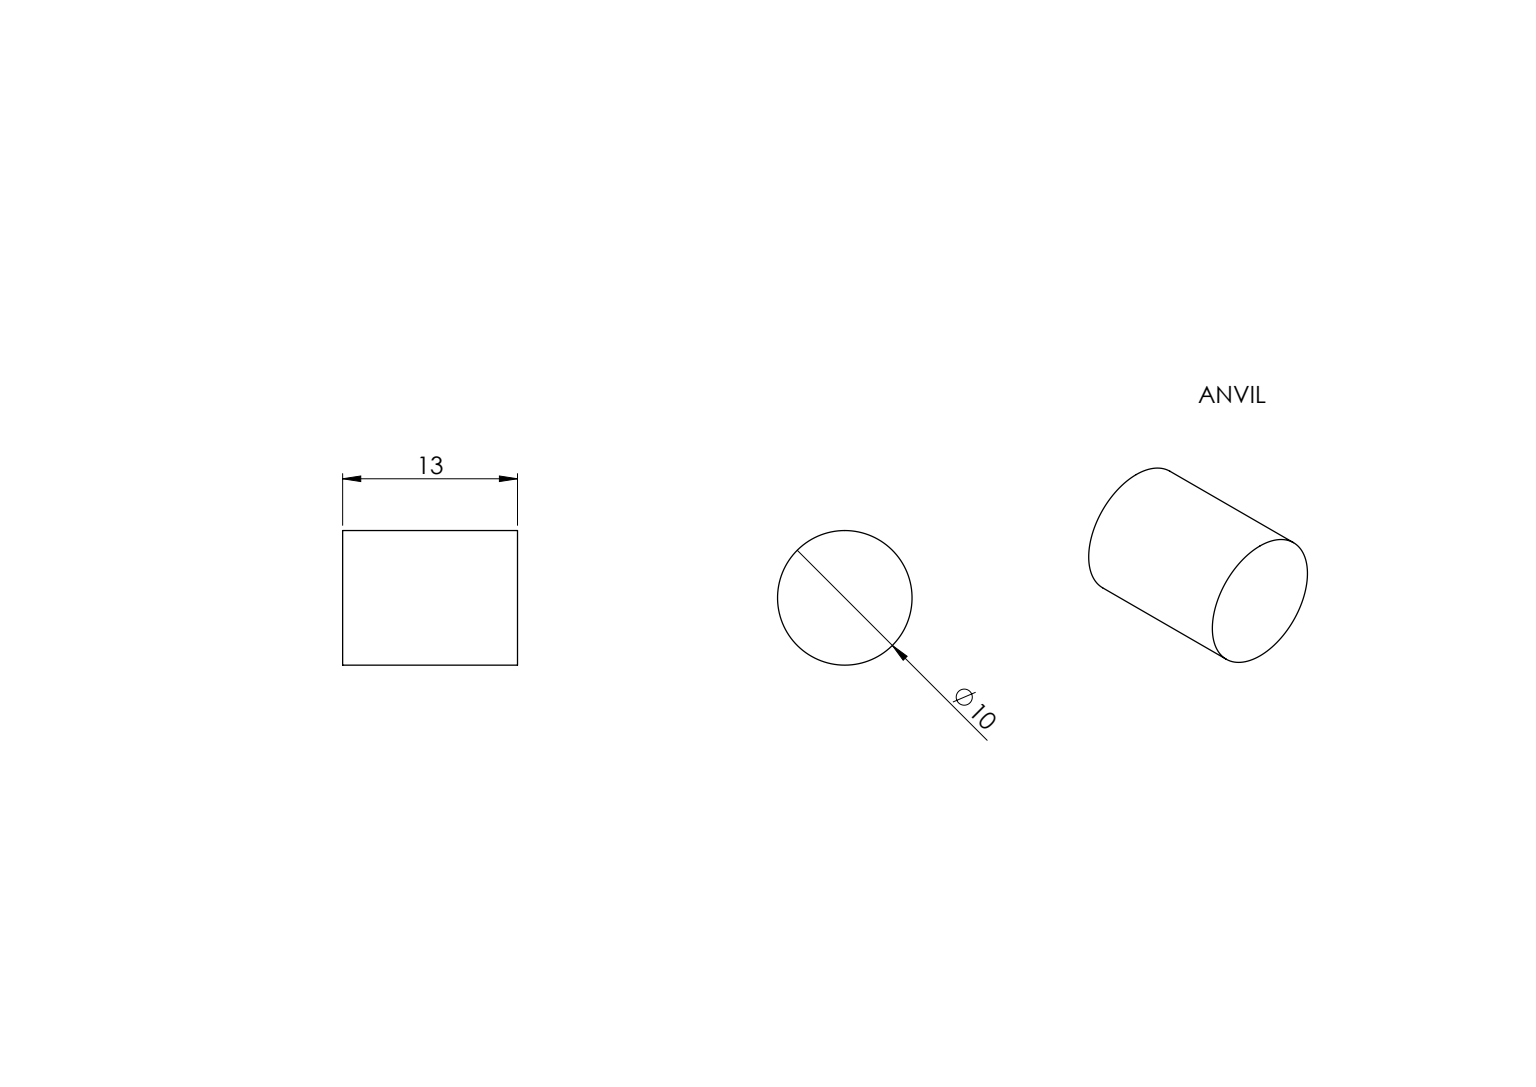
ISO-10303-21;
HEADER;
FILE_DESCRIPTION (('STEP AP214'),
    '1' );
FILE_NAME ('anvil.step',
    '2026-10-22T12:35:56',
    ( '' ),
    ( '' ),
    'SwSTEP 2.0',
    'SolidWorks 2026',
    '' );
FILE_SCHEMA (( 'AUTOMOTIVE_DESIGN' ));
ENDSEC;

DATA;
#84=AXIS2_PLACEMENT_3D ( 'NONE', #1775, #288, #1276 ) ;
#101=EDGE_CURVE ( 'NONE', #738, #770, #2722, .T. ) ;
#112=CLOSED_SHELL ( 'NONE', ( #233, #2010, #1720, #1045 ) ) ;
#119=PRODUCT_DEFINITION_SHAPE ( 'NONE', 'NONE',  #694 ) ;
#122=MECHANICAL_DESIGN_GEOMETRIC_PRESENTATION_REPRESENTATION('',(#1113),#303);
#125=EDGE_LOOP ( 'NONE', ( #1383, #1724 ) ) ;
#153=DIRECTION ( 'NONE',  ( -1.000000000000000000, -2.312964634635742957E-16, -0.000000000000000000 ) ) ;
#179=DIRECTION ( 'NONE',  ( -2.312964634635742957E-16, 1.000000000000000000, 0.000000000000000000 ) ) ;
#233=ADVANCED_FACE ( 'NONE', ( #2687 ), #1203, .T. ) ;
#234=EDGE_CURVE ( 'NONE', #516, #770, #260, .T. ) ;
#242=CARTESIAN_POINT ( 'NONE',  ( -23.99999999999999645, 4.999999999999993783, 7.500000000000000888 ) ) ;
#256=CARTESIAN_POINT ( 'NONE',  ( -37.00000000000000000, -9.935696797193021379E-15, 7.500000000000000000 ) ) ;
#260=LINE ( 'NONE', #242, #2360 ) ;
#284=AXIS2_PLACEMENT_3D ( 'NONE', #1975, #461, #492 ) ;
#285=VECTOR ( 'NONE', #856, 1000.000000000000000 ) ;
#288=DIRECTION ( 'NONE',  ( 1.000000000000000000, 2.312964634635742957E-16, 0.000000000000000000 ) ) ;
#303=( GEOMETRIC_REPRESENTATION_CONTEXT ( 3 ) GLOBAL_UNCERTAINTY_ASSIGNED_CONTEXT ( ( #2916 ) ) GLOBAL_UNIT_ASSIGNED_CONTEXT ( ( #3088, #2138, #2843 ) ) REPRESENTATION_CONTEXT ( 'NONE', 'WORKASPACE' ) );
#307=PRODUCT_DEFINITION_CONTEXT ( 'detailed design', #2566, 'design' ) ;
#374=CARTESIAN_POINT ( 'NONE',  ( -23.99999999999999645, -6.928842772166554697E-15, 7.500000000000000000 ) ) ;
#380=UNCERTAINTY_MEASURE_WITH_UNIT (LENGTH_MEASURE( 1.000000000000000082E-05 ), #1214, 'distance_accuracy_value', 'NONE');
#437=PRODUCT_CONTEXT ( 'NONE', #1344, 'mechanical' ) ;
#441=( NAMED_UNIT ( * ) SI_UNIT ( $, .STERADIAN. ) SOLID_ANGLE_UNIT ( ) );
#444=UNCERTAINTY_MEASURE_WITH_UNIT (LENGTH_MEASURE( 1.000000000000000082E-05 ), #3138, 'distance_accuracy_value', 'NONE');
#461=DIRECTION ( 'NONE',  ( -1.000000000000000000, -2.312964634635742957E-16, -0.000000000000000000 ) ) ;
#492=DIRECTION ( 'NONE',  ( 0.000000000000000000, -1.000000000000000000, 0.000000000000000000 ) ) ;
#516=VERTEX_POINT ( 'NONE', #608 ) ;
#523=ORIENTED_EDGE ( 'NONE', *, *, #2382, .F. ) ;
#541=LINE ( 'NONE', #1281, #285 ) ;
#544=CYLINDRICAL_SURFACE ( 'NONE', #1147, 5.000000000000000888 ) ;
#548=VERTEX_POINT ( 'NONE', #831 ) ;
#578=CIRCLE ( 'NONE', #2085, 5.000000000000000888 ) ;
#608=CARTESIAN_POINT ( 'NONE',  ( -23.99999999999999645, 4.999999999999994671, 7.500000000000000888 ) ) ;
#634=ORIENTED_EDGE ( 'NONE', *, *, #1634, .T. ) ;
#656=SHAPE_REPRESENTATION_RELATIONSHIP ( 'NONE' , 'NONE' ,  #1116, #1362 ) ;
#694=PRODUCT_DEFINITION ( 'UNKNOWN', '', #708, #307 ) ;
#705=COLOUR_RGB ( '',0.8941176470588234615, 0.8941176470588234615, 0.8941176470588234615 ) ;
#708=PRODUCT_DEFINITION_FORMATION_WITH_SPECIFIED_SOURCE ( 'ANY', '', #2285, .NOT_KNOWN. ) ;
#731=EDGE_CURVE ( 'NONE', #548, #738, #541, .T. ) ;
#738=VERTEX_POINT ( 'NONE', #1122 ) ;
#744=PLANE ( 'NONE',  #1838 ) ;
#770=VERTEX_POINT ( 'NONE', #1596 ) ;
#831=CARTESIAN_POINT ( 'NONE',  ( -23.99999999999999645, -5.000000000000007994, 7.500000000000000000 ) ) ;
#841=EDGE_LOOP ( 'NONE', ( #929, #2082, #634, #2585 ) ) ;
#856=DIRECTION ( 'NONE',  ( -1.000000000000000000, -2.312964634635742957E-16, -0.000000000000000000 ) ) ;
#881=STYLED_ITEM('',(#3250),#2099);
#929=ORIENTED_EDGE ( 'NONE', *, *, #1865, .F. ) ;
#946=ORIENTED_EDGE ( 'NONE', *, *, #234, .F. ) ;
#952=SHAPE_DEFINITION_REPRESENTATION ( #119, #1116 ) ;
#1020=CARTESIAN_POINT ( 'NONE',  ( -23.99999999999999645, -6.928842772166554697E-15, 7.500000000000000000 ) ) ;
#1045=ADVANCED_FACE ( 'NONE', ( #2749 ), #744, .F. ) ;
#1091=CARTESIAN_POINT ( 'NONE',  ( -23.99999999999999645, -6.928842772166554697E-15, 7.500000000000000000 ) ) ;
#1098=PRESENTATION_STYLE_ASSIGNMENT (( #2876 ) ) ;
#1113=STYLED_ITEM ( 'NONE', ( #1098 ), #1362 ) ;
#1116=SHAPE_REPRESENTATION ( 'anvil', ( #2878 ), #2622 ) ;
#1122=CARTESIAN_POINT ( 'NONE',  ( -37.00000000000000000, -5.000000000000010658, 7.500000000000000000 ) ) ;
#1147=AXIS2_PLACEMENT_3D ( 'NONE', #374, #153, #2286 ) ;
#1203=CYLINDRICAL_SURFACE ( 'NONE', #284, 5.000000000000000888 ) ;
#1214=( LENGTH_UNIT ( ) NAMED_UNIT ( * ) SI_UNIT ( .MILLI., .METRE. ) );
#1276=DIRECTION ( 'NONE',  ( 0.000000000000000000, 1.000000000000000000, 0.000000000000000000 ) ) ;
#1281=CARTESIAN_POINT ( 'NONE',  ( -23.99999999999999645, -5.000000000000007994, 7.500000000000000000 ) ) ;
#1344=APPLICATION_CONTEXT ( 'automotive_design' ) ;
#1362=ADVANCED_BREP_SHAPE_REPRESENTATION ( '', ( #2099, #2878 ), #2622 ) ;
#1364=DIRECTION ( 'NONE',  ( 0.000000000000000000, 1.000000000000000000, 0.000000000000000000 ) ) ;
#1383=ORIENTED_EDGE ( 'NONE', *, *, #2382, .T. ) ;
#1394=FACE_OUTER_BOUND ( 'NONE', #2795, .T. ) ;
#1466=DIRECTION ( 'NONE',  ( 1.000000000000000000, 2.312964634635742957E-16, 0.000000000000000000 ) ) ;
#1499=CIRCLE ( 'NONE', #84, 5.000000000000000888 ) ;
#1566=( GEOMETRIC_REPRESENTATION_CONTEXT ( 3 ) GLOBAL_UNCERTAINTY_ASSIGNED_CONTEXT ( ( #380 ) ) GLOBAL_UNIT_ASSIGNED_CONTEXT ( ( #1214, #1717, #2699 ) ) REPRESENTATION_CONTEXT ( 'NONE', 'WORKASPACE' ) );
#1596=CARTESIAN_POINT ( 'NONE',  ( -37.00000000000000000, 4.999999999999991118, 7.500000000000000888 ) ) ;
#1634=EDGE_CURVE ( 'NONE', #770, #738, #1499, .T. ) ;
#1638=FACE_OUTER_BOUND ( 'NONE', #125, .T. ) ;
#1672=CARTESIAN_POINT ( 'NONE',  ( -37.00000000000000000, -9.935696797193021379E-15, 7.500000000000000000 ) ) ;
#1697=AXIS2_PLACEMENT_3D ( 'NONE', #1091, #2586, #2836 ) ;
#1717=( NAMED_UNIT ( * ) PLANE_ANGLE_UNIT ( ) SI_UNIT ( $, .RADIAN. ) );
#1720=ADVANCED_FACE ( 'NONE', ( #1638 ), #2157, .T. ) ;
#1724=ORIENTED_EDGE ( 'NONE', *, *, #1865, .T. ) ;
#1775=CARTESIAN_POINT ( 'NONE',  ( -37.00000000000000000, -9.935696797193021379E-15, 7.500000000000000000 ) ) ;
#1837=DIRECTION ( 'NONE',  ( 1.000000000000000000, 0.000000000000000000, 0.000000000000000000 ) ) ;
#1838=AXIS2_PLACEMENT_3D ( 'NONE', #256, #2515, #3043 ) ;
#1865=EDGE_CURVE ( 'NONE', #516, #548, #578, .T. ) ;
#1881=MECHANICAL_DESIGN_GEOMETRIC_PRESENTATION_REPRESENTATION('',(#881),#1566);
#1975=CARTESIAN_POINT ( 'NONE',  ( -23.99999999999999645, -6.928842772166554697E-15, 7.500000000000000000 ) ) ;
#1992=DIRECTION ( 'NONE',  ( 0.000000000000000000, 1.000000000000000000, 0.000000000000000000 ) ) ;
#2010=ADVANCED_FACE ( 'NONE', ( #1394 ), #544, .T. ) ;
#2082=ORIENTED_EDGE ( 'NONE', *, *, #234, .T. ) ;
#2085=AXIS2_PLACEMENT_3D ( 'NONE', #1020, #1466, #1992 ) ;
#2087=ORIENTED_EDGE ( 'NONE', *, *, #101, .F. ) ;
#2099=MANIFOLD_SOLID_BREP ( 'Boss-Extrude1', #112 ) ;
#2101=SURFACE_SIDE_STYLE ('',( #3156 ) ) ;
#2138=( NAMED_UNIT ( * ) PLANE_ANGLE_UNIT ( ) SI_UNIT ( $, .RADIAN. ) );
#2157=PLANE ( 'NONE',  #2694 ) ;
#2208=ORIENTED_EDGE ( 'NONE', *, *, #1634, .F. ) ;
#2285=PRODUCT ( 'anvil', 'anvil', '', ( #437 ) ) ;
#2286=DIRECTION ( 'NONE',  ( 0.000000000000000000, -1.000000000000000000, 0.000000000000000000 ) ) ;
#2312=AXIS2_PLACEMENT_3D ( 'NONE', #1672, #3142, #1364 ) ;
#2360=VECTOR ( 'NONE', #3193, 1000.000000000000000 ) ;
#2382=EDGE_CURVE ( 'NONE', #548, #516, #2982, .T. ) ;
#2409=DIRECTION ( 'NONE',  ( 1.000000000000000000, 2.312964634635742957E-16, 0.000000000000000000 ) ) ;
#2421=FILL_AREA_STYLE_COLOUR ( '', #705 ) ;
#2515=DIRECTION ( 'NONE',  ( 1.000000000000000000, 2.312964634635742957E-16, 0.000000000000000000 ) ) ;
#2537=ORIENTED_EDGE ( 'NONE', *, *, #731, .T. ) ;
#2566=APPLICATION_CONTEXT ( 'automotive_design' ) ;
#2585=ORIENTED_EDGE ( 'NONE', *, *, #731, .F. ) ;
#2586=DIRECTION ( 'NONE',  ( 1.000000000000000000, 2.312964634635742957E-16, 0.000000000000000000 ) ) ;
#2622=( GEOMETRIC_REPRESENTATION_CONTEXT ( 3 ) GLOBAL_UNCERTAINTY_ASSIGNED_CONTEXT ( ( #444 ) ) GLOBAL_UNIT_ASSIGNED_CONTEXT ( ( #3138, #2664, #441 ) ) REPRESENTATION_CONTEXT ( 'NONE', 'WORKASPACE' ) );
#2648=FILL_AREA_STYLE ('',( #2421 ) ) ;
#2664=( NAMED_UNIT ( * ) PLANE_ANGLE_UNIT ( ) SI_UNIT ( $, .RADIAN. ) );
#2687=FACE_OUTER_BOUND ( 'NONE', #841, .T. ) ;
#2694=AXIS2_PLACEMENT_3D ( 'NONE', #3144, #2409, #179 ) ;
#2699=( NAMED_UNIT ( * ) SI_UNIT ( $, .STERADIAN. ) SOLID_ANGLE_UNIT ( ) );
#2722=CIRCLE ( 'NONE', #2312, 5.000000000000000888 ) ;
#2749=FACE_OUTER_BOUND ( 'NONE', #2781, .T. ) ;
#2781=EDGE_LOOP ( 'NONE', ( #2087, #2208 ) ) ;
#2795=EDGE_LOOP ( 'NONE', ( #946, #523, #2537, #2840 ) ) ;
#2799=DIRECTION ( 'NONE',  ( 0.000000000000000000, 0.000000000000000000, 1.000000000000000000 ) ) ;
#2836=DIRECTION ( 'NONE',  ( 0.000000000000000000, 1.000000000000000000, 0.000000000000000000 ) ) ;
#2840=ORIENTED_EDGE ( 'NONE', *, *, #101, .T. ) ;
#2843=( NAMED_UNIT ( * ) SI_UNIT ( $, .STERADIAN. ) SOLID_ANGLE_UNIT ( ) );
#2876=SURFACE_STYLE_USAGE ( .BOTH. , #2101 ) ;
#2878=AXIS2_PLACEMENT_3D ( 'NONE', #3071, #2799, #1837 ) ;
#2916=UNCERTAINTY_MEASURE_WITH_UNIT (LENGTH_MEASURE( 1.000000000000000082E-05 ), #3088, 'distance_accuracy_value', 'NONE');
#2982=CIRCLE ( 'NONE', #1697, 5.000000000000000888 ) ;
#3043=DIRECTION ( 'NONE',  ( -2.312964634635742957E-16, 1.000000000000000000, 0.000000000000000000 ) ) ;
#3071=CARTESIAN_POINT ( 'NONE',  ( 0.000000000000000000, 0.000000000000000000, 0.000000000000000000 ) ) ;
#3088=( LENGTH_UNIT ( ) NAMED_UNIT ( * ) SI_UNIT ( .MILLI., .METRE. ) );
#3138=( LENGTH_UNIT ( ) NAMED_UNIT ( * ) SI_UNIT ( .MILLI., .METRE. ) );
#3142=DIRECTION ( 'NONE',  ( 1.000000000000000000, 2.312964634635742957E-16, 0.000000000000000000 ) ) ;
#3144=CARTESIAN_POINT ( 'NONE',  ( -23.99999999999999645, -6.928842772166554697E-15, 7.500000000000000000 ) ) ;
#3156=SURFACE_STYLE_FILL_AREA ( #2648 ) ;
#3193=DIRECTION ( 'NONE',  ( -1.000000000000000000, -2.312964634635742957E-16, -0.000000000000000000 ) ) ;
#3244=COLOUR_RGB('Sky Blue',0.24,0.69,0.87);
#3245=FILL_AREA_STYLE_COLOUR('',#3244);
#3246=FILL_AREA_STYLE('',(#3245));
#3247=SURFACE_STYLE_FILL_AREA(#3246);
#3248=SURFACE_SIDE_STYLE('',(#3247));
#3249=SURFACE_STYLE_USAGE(.BOTH.,#3248);
#3250=PRESENTATION_STYLE_ASSIGNMENT((#3249));
ENDSEC;
END-ISO-10303-21;
